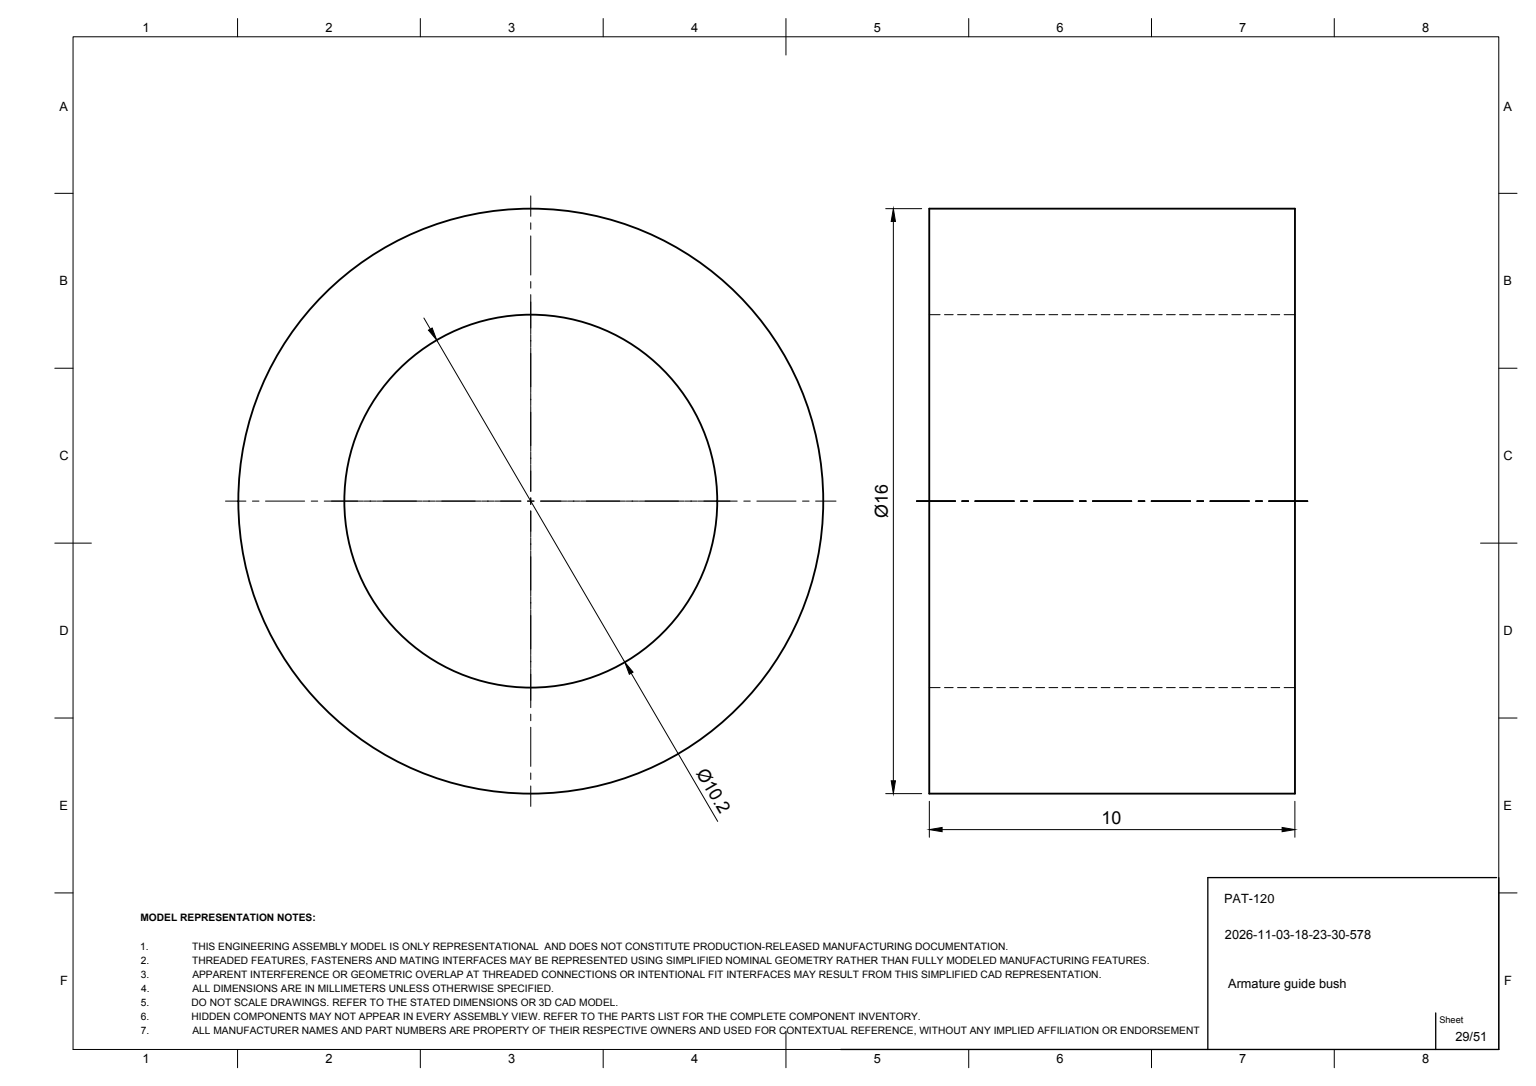
ISO-10303-21;
HEADER;
/* Generated by software containing ST-Developer
 * from STEP Tools, Inc. (www.steptools.com) 
 */

FILE_DESCRIPTION(
/* description */ ('Vibration shaker table dummy'),
/* implementation_level */ '2;1');

FILE_NAME(
/* name */ 'Armature guide bush.step',
/* time_stamp */ '2026-10-27T10:55:14-07:00',
/* author */ (''),
/* organization */ (''),
/* preprocessor_version */ 'ST-DEVELOPER v20.2',
/* originating_system */ 'Autodesk Translation Framework v15.17.0.0',
/* authorisation */ '');

FILE_SCHEMA (('AUTOMOTIVE_DESIGN { 1 0 10303 214 3 1 1 }'));
ENDSEC;

DATA;
#10=MECHANICAL_DESIGN_GEOMETRIC_PRESENTATION_REPRESENTATION('',(#710),#22394);
#618=SHAPE_REPRESENTATION_RELATIONSHIP('SRR','None',#22664,#664);
#664=ADVANCED_BREP_SHAPE_REPRESENTATION('',(#756),#22370);
#710=STYLED_ITEM('',(#22947),#756);
#756=MANIFOLD_SOLID_BREP('Body1',#9228);
#941=FACE_BOUND('',#2264,.T.);
#942=FACE_BOUND('',#2266,.T.);
#1210=PLANE('',#10273);
#1211=PLANE('',#10274);
#1597=FACE_OUTER_BOUND('',#2261,.T.);
#1598=FACE_OUTER_BOUND('',#2262,.T.);
#1599=FACE_OUTER_BOUND('',#2263,.T.);
#1600=FACE_OUTER_BOUND('',#2265,.T.);
#2261=EDGE_LOOP('',(#7410,#7411,#7412,#7413));
#2262=EDGE_LOOP('',(#7414,#7415,#7416,#7417));
#2263=EDGE_LOOP('',(#7418));
#2264=EDGE_LOOP('',(#7419));
#2265=EDGE_LOOP('',(#7420));
#2266=EDGE_LOOP('',(#7421));
#2972=LINE('',#20984,#3591);
#2973=LINE('',#20990,#3592);
#3591=VECTOR('',#12318,0.51);
#3592=VECTOR('',#12325,0.8);
#4088=CIRCLE('',#10268,0.51);
#4089=CIRCLE('',#10269,0.51);
#4090=CIRCLE('',#10271,0.8);
#4091=CIRCLE('',#10272,0.8);
#4755=VERTEX_POINT('',#20981);
#4756=VERTEX_POINT('',#20983);
#4757=VERTEX_POINT('',#20987);
#4758=VERTEX_POINT('',#20989);
#5698=EDGE_CURVE('',#4755,#4755,#4088,.T.);
#5699=EDGE_CURVE('',#4755,#4756,#2972,.T.);
#5700=EDGE_CURVE('',#4756,#4756,#4089,.T.);
#5701=EDGE_CURVE('',#4757,#4757,#4090,.T.);
#5702=EDGE_CURVE('',#4757,#4758,#2973,.T.);
#5703=EDGE_CURVE('',#4758,#4758,#4091,.T.);
#7410=ORIENTED_EDGE('',*,*,#5698,.F.);
#7411=ORIENTED_EDGE('',*,*,#5699,.T.);
#7412=ORIENTED_EDGE('',*,*,#5700,.T.);
#7413=ORIENTED_EDGE('',*,*,#5699,.F.);
#7414=ORIENTED_EDGE('',*,*,#5701,.F.);
#7415=ORIENTED_EDGE('',*,*,#5702,.T.);
#7416=ORIENTED_EDGE('',*,*,#5703,.T.);
#7417=ORIENTED_EDGE('',*,*,#5702,.F.);
#7418=ORIENTED_EDGE('',*,*,#5701,.T.);
#7419=ORIENTED_EDGE('',*,*,#5698,.T.);
#7420=ORIENTED_EDGE('',*,*,#5703,.F.);
#7421=ORIENTED_EDGE('',*,*,#5700,.F.);
#8608=CYLINDRICAL_SURFACE('',#10267,0.51);
#8609=CYLINDRICAL_SURFACE('',#10270,0.8);
#8962=ADVANCED_FACE('',(#1597),#8608,.F.);
#8963=ADVANCED_FACE('',(#1598),#8609,.T.);
#8964=ADVANCED_FACE('',(#1599,#941),#1210,.T.);
#8965=ADVANCED_FACE('',(#1600,#942),#1211,.F.);
#9228=CLOSED_SHELL('',(#8962,#8963,#8964,#8965));
#10266=AXIS2_PLACEMENT_3D('',#20979,#12312,#12313);
#10267=AXIS2_PLACEMENT_3D('',#20980,#12314,#12315);
#10268=AXIS2_PLACEMENT_3D('',#20982,#12316,#12317);
#10269=AXIS2_PLACEMENT_3D('',#20985,#12319,#12320);
#10270=AXIS2_PLACEMENT_3D('',#20986,#12321,#12322);
#10271=AXIS2_PLACEMENT_3D('',#20988,#12323,#12324);
#10272=AXIS2_PLACEMENT_3D('',#20991,#12326,#12327);
#10273=AXIS2_PLACEMENT_3D('',#20992,#12328,#12329);
#10274=AXIS2_PLACEMENT_3D('',#20993,#12330,#12331);
#12312=DIRECTION('axis',(0.,0.,1.));
#12313=DIRECTION('refdir',(1.,0.,0.));
#12314=DIRECTION('center_axis',(0.,0.,1.));
#12315=DIRECTION('ref_axis',(1.,0.,0.));
#12316=DIRECTION('center_axis',(0.,0.,-1.));
#12317=DIRECTION('ref_axis',(1.,0.,0.));
#12318=DIRECTION('',(0.,0.,-1.));
#12319=DIRECTION('center_axis',(0.,0.,-1.));
#12320=DIRECTION('ref_axis',(1.,0.,0.));
#12321=DIRECTION('center_axis',(0.,0.,1.));
#12322=DIRECTION('ref_axis',(1.,0.,0.));
#12323=DIRECTION('center_axis',(0.,0.,1.));
#12324=DIRECTION('ref_axis',(1.,0.,0.));
#12325=DIRECTION('',(0.,0.,-1.));
#12326=DIRECTION('center_axis',(0.,0.,1.));
#12327=DIRECTION('ref_axis',(1.,0.,0.));
#12328=DIRECTION('center_axis',(0.,0.,1.));
#12329=DIRECTION('ref_axis',(1.,0.,0.));
#12330=DIRECTION('center_axis',(0.,0.,1.));
#12331=DIRECTION('ref_axis',(1.,0.,0.));
#20979=CARTESIAN_POINT('',(0.,0.,0.));
#20980=CARTESIAN_POINT('Origin',(0.,0.,9.));
#20981=CARTESIAN_POINT('',(-0.51,-6.2456986756515E-17,10.));
#20982=CARTESIAN_POINT('Origin',(0.,0.,10.));
#20983=CARTESIAN_POINT('',(-0.51,-6.2456986756515E-17,9.));
#20984=CARTESIAN_POINT('',(-0.51,-6.2456986756515E-17,9.));
#20985=CARTESIAN_POINT('Origin',(0.,0.,9.));
#20986=CARTESIAN_POINT('Origin',(0.,0.,9.));
#20987=CARTESIAN_POINT('',(-0.8,-9.79717439317883E-17,10.));
#20988=CARTESIAN_POINT('Origin',(0.,0.,10.));
#20989=CARTESIAN_POINT('',(-0.8,-9.79717439317883E-17,9.));
#20990=CARTESIAN_POINT('',(-0.8,-9.79717439317883E-17,9.));
#20991=CARTESIAN_POINT('Origin',(0.,0.,9.));
#20992=CARTESIAN_POINT('Origin',(0.,0.,10.));
#20993=CARTESIAN_POINT('Origin',(0.,0.,9.));
#22319=UNCERTAINTY_MEASURE_WITH_UNIT(LENGTH_MEASURE(0.001),#22395,
'DISTANCE_ACCURACY_VALUE',
'Maximum model space distance between geometric entities at asserted c
onnectivities');
#22343=UNCERTAINTY_MEASURE_WITH_UNIT(LENGTH_MEASURE(0.001),#22395,
'DISTANCE_ACCURACY_VALUE',
'Maximum model space distance between geometric entities at asserted c
onnectivities');
#22370=(
GEOMETRIC_REPRESENTATION_CONTEXT(3)
GLOBAL_UNCERTAINTY_ASSIGNED_CONTEXT((#22319))
GLOBAL_UNIT_ASSIGNED_CONTEXT((#22395,#22397,#22398))
REPRESENTATION_CONTEXT('','3D')
);
#22394=(
GEOMETRIC_REPRESENTATION_CONTEXT(3)
GLOBAL_UNCERTAINTY_ASSIGNED_CONTEXT((#22343))
GLOBAL_UNIT_ASSIGNED_CONTEXT((#22395,#22397,#22398))
REPRESENTATION_CONTEXT('','3D')
);
#22395=(
LENGTH_UNIT()
NAMED_UNIT(*)
SI_UNIT(.CENTI.,.METRE.)
);
#22397=(
NAMED_UNIT(*)
PLANE_ANGLE_UNIT()
SI_UNIT($,.RADIAN.)
);
#22398=(
NAMED_UNIT(*)
SI_UNIT($,.STERADIAN.)
SOLID_ANGLE_UNIT()
);
#22425=SHAPE_DEFINITION_REPRESENTATION(#22475,#22664);
#22475=PRODUCT_DEFINITION_SHAPE('',$,#22715);
#22664=SHAPE_REPRESENTATION('',(#10266),#22370);
#22688=PRODUCT_DEFINITION_CONTEXT('part definition',#22840,'design');
#22715=PRODUCT_DEFINITION('Armature guide bush','Armature guide bush',#22765,
#22688);
#22765=PRODUCT_DEFINITION_FORMATION('',$,#22868);
#22840=APPLICATION_CONTEXT(
'Core Data for Automotive Mechanical Design Process');
#22841=PRODUCT_CONTEXT('part definition',#22840,'mechanical');
#22868=PRODUCT('Armature guide bush','Armature guide bush',
'Armature guide bush',(#22841));
#22941=COLOUR_RGB('Light Blue',0.38,0.62,0.78);
#22942=FILL_AREA_STYLE_COLOUR('',#22941);
#22943=FILL_AREA_STYLE('',(#22942));
#22944=SURFACE_STYLE_FILL_AREA(#22943);
#22945=SURFACE_SIDE_STYLE('',(#22944));
#22946=SURFACE_STYLE_USAGE(.BOTH.,#22945);
#22947=PRESENTATION_STYLE_ASSIGNMENT((#22946));
ENDSEC;
END-ISO-10303-21;
